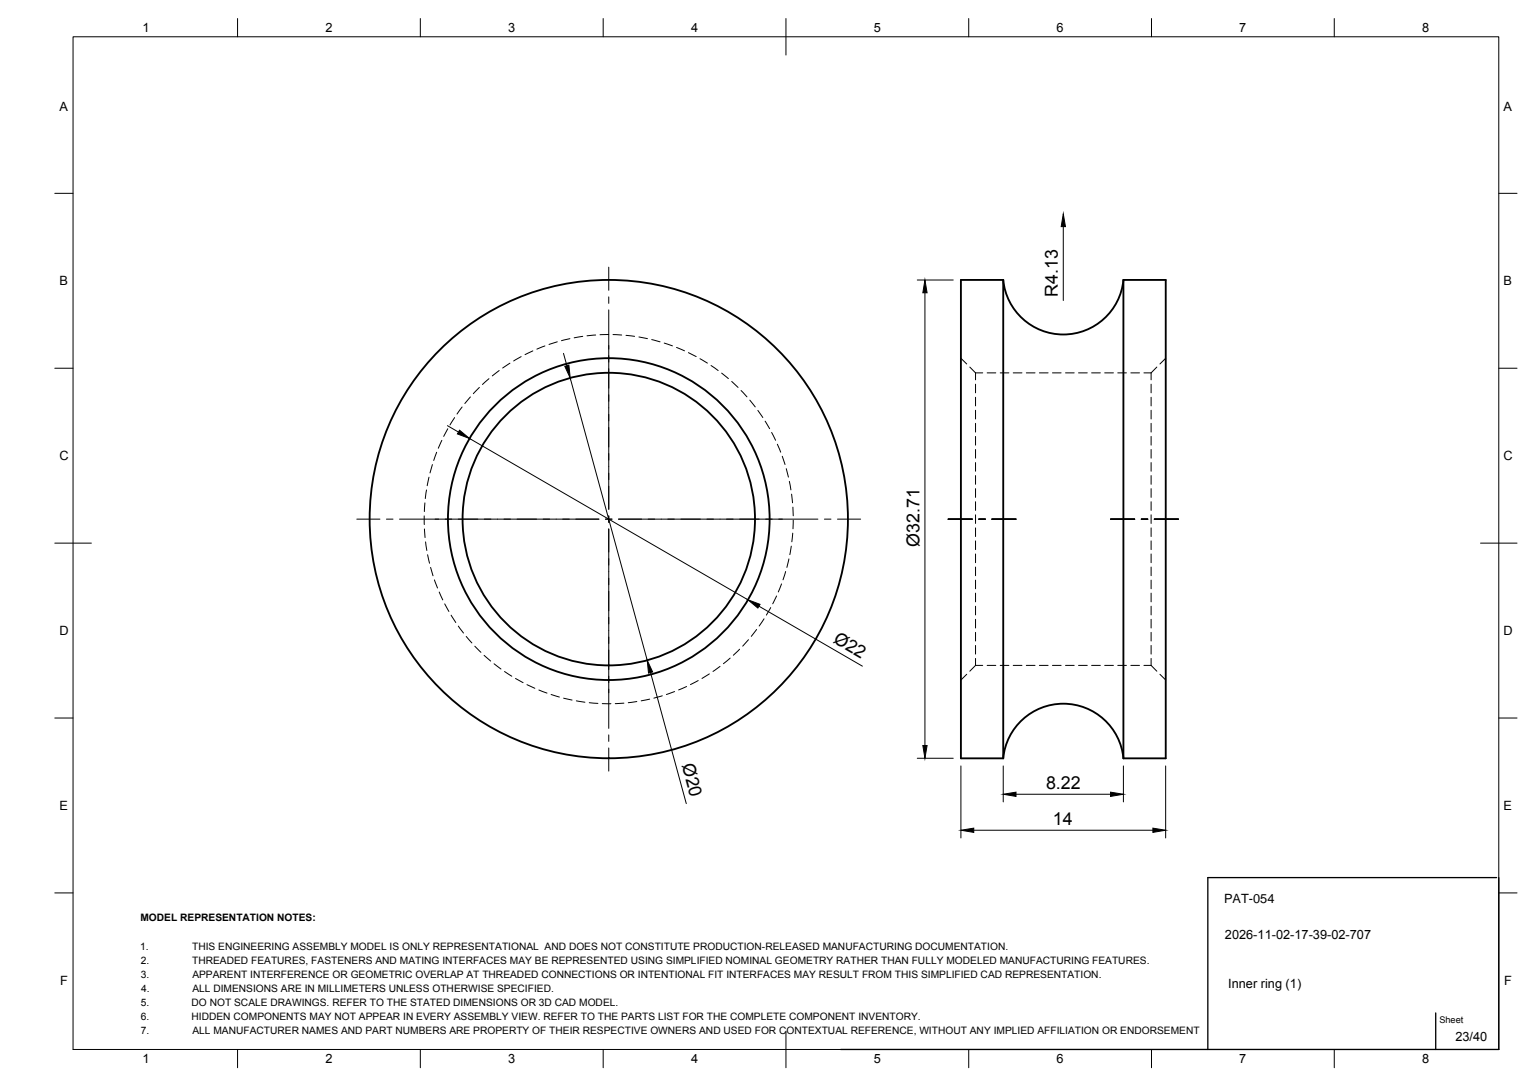
ISO-10303-21;
HEADER;
/* Generated by software containing ST-Developer
 * from STEP Tools, Inc. (www.steptools.com) 
 */

FILE_DESCRIPTION(
/* description */ ('PAT-054'),
/* implementation_level */ '2;1');

FILE_NAME(
/* name */ 'Inner ring (1).step',
/* time_stamp */ '2026-10-29T16:38:13-07:00',
/* author */ (''),
/* organization */ (''),
/* preprocessor_version */ 'ST-DEVELOPER v20.2',
/* originating_system */ 'Autodesk Translation Framework v15.17.0.0',
/* authorisation */ '');

FILE_SCHEMA (('AUTOMOTIVE_DESIGN { 1 0 10303 214 3 1 1 }'));
ENDSEC;

DATA;
#10=MECHANICAL_DESIGN_GEOMETRIC_PRESENTATION_REPRESENTATION('',(#920),#33981);
#781=CONICAL_SURFACE('',#14012,1.05,0.785398163397449);
#782=CONICAL_SURFACE('',#14019,1.05,0.785398163397449);
#809=TOROIDAL_SURFACE('',#14001,1.675,0.412776);
#825=SHAPE_REPRESENTATION_RELATIONSHIP('SRR','None',#34200,#869);
#869=ADVANCED_BREP_SHAPE_REPRESENTATION('',(#979),#33948);
#920=STYLED_ITEM('',(#34517),#979);
#979=MANIFOLD_SOLID_BREP('Body1',#13031);
#1137=FACE_BOUND('',#2629,.T.);
#1138=FACE_BOUND('',#2632,.T.);
#1327=PLANE('',#14014);
#1328=PLANE('',#14017);
#1776=FACE_OUTER_BOUND('',#2624,.T.);
#1777=FACE_OUTER_BOUND('',#2625,.T.);
#1778=FACE_OUTER_BOUND('',#2626,.T.);
#1779=FACE_OUTER_BOUND('',#2627,.T.);
#1780=FACE_OUTER_BOUND('',#2628,.T.);
#1781=FACE_OUTER_BOUND('',#2630,.T.);
#1782=FACE_OUTER_BOUND('',#2631,.T.);
#1783=FACE_OUTER_BOUND('',#2633,.T.);
#2624=EDGE_LOOP('',(#9425,#9426,#9427,#9428,#9429,#9430));
#2625=EDGE_LOOP('',(#9431,#9432,#9433,#9434,#9435));
#2626=EDGE_LOOP('',(#9436,#9437,#9438,#9439));
#2627=EDGE_LOOP('',(#9440,#9441,#9442,#9443));
#2628=EDGE_LOOP('',(#9444));
#2629=EDGE_LOOP('',(#9445));
#2630=EDGE_LOOP('',(#9446,#9447,#9448,#9449,#9450));
#2631=EDGE_LOOP('',(#9451));
#2632=EDGE_LOOP('',(#9452));
#2633=EDGE_LOOP('',(#9453,#9454,#9455,#9456));
#3474=LINE('',#19805,#4408);
#3475=LINE('',#19811,#4409);
#3476=LINE('',#19815,#4410);
#3477=LINE('',#19821,#4411);
#3478=LINE('',#19826,#4412);
#4408=VECTOR('',#16025,1.63531);
#4409=VECTOR('',#16032,1.);
#4410=VECTOR('',#16037,1.05);
#4411=VECTOR('',#16046,1.63531);
#4412=VECTOR('',#16053,1.05);
#5322=CIRCLE('',#14002,1.63531);
#5323=CIRCLE('',#14003,1.63531);
#5324=CIRCLE('',#14004,0.412776);
#5325=CIRCLE('',#14005,1.63531);
#5326=CIRCLE('',#14006,1.63531);
#5327=CIRCLE('',#14008,1.63531);
#5328=CIRCLE('',#14010,1.);
#5329=CIRCLE('',#14011,1.);
#5330=CIRCLE('',#14013,1.1);
#5331=CIRCLE('',#14016,1.63531);
#5332=CIRCLE('',#14018,1.1);
#5890=VERTEX_POINT('',#19794);
#5891=VERTEX_POINT('',#19795);
#5892=VERTEX_POINT('',#19798);
#5893=VERTEX_POINT('',#19800);
#5894=VERTEX_POINT('',#19804);
#5895=VERTEX_POINT('',#19808);
#5896=VERTEX_POINT('',#19810);
#5897=VERTEX_POINT('',#19814);
#5898=VERTEX_POINT('',#19819);
#5899=VERTEX_POINT('',#19823);
#7212=EDGE_CURVE('',#5890,#5891,#5322,.T.);
#7213=EDGE_CURVE('',#5891,#5890,#5323,.T.);
#7214=EDGE_CURVE('',#5891,#5892,#5324,.T.);
#7215=EDGE_CURVE('',#5893,#5892,#5325,.T.);
#7216=EDGE_CURVE('',#5892,#5893,#5326,.T.);
#7217=EDGE_CURVE('',#5893,#5894,#3474,.T.);
#7218=EDGE_CURVE('',#5894,#5894,#5327,.T.);
#7219=EDGE_CURVE('',#5895,#5895,#5328,.T.);
#7220=EDGE_CURVE('',#5895,#5896,#3475,.T.);
#7221=EDGE_CURVE('',#5896,#5896,#5329,.T.);
#7222=EDGE_CURVE('',#5896,#5897,#3476,.T.);
#7223=EDGE_CURVE('',#5897,#5897,#5330,.T.);
#7224=EDGE_CURVE('',#5898,#5898,#5331,.T.);
#7225=EDGE_CURVE('',#5898,#5890,#3477,.T.);
#7226=EDGE_CURVE('',#5899,#5899,#5332,.T.);
#7227=EDGE_CURVE('',#5899,#5895,#3478,.T.);
#9425=ORIENTED_EDGE('',*,*,#7212,.F.);
#9426=ORIENTED_EDGE('',*,*,#7213,.F.);
#9427=ORIENTED_EDGE('',*,*,#7214,.T.);
#9428=ORIENTED_EDGE('',*,*,#7215,.F.);
#9429=ORIENTED_EDGE('',*,*,#7216,.F.);
#9430=ORIENTED_EDGE('',*,*,#7214,.F.);
#9431=ORIENTED_EDGE('',*,*,#7215,.T.);
#9432=ORIENTED_EDGE('',*,*,#7216,.T.);
#9433=ORIENTED_EDGE('',*,*,#7217,.T.);
#9434=ORIENTED_EDGE('',*,*,#7218,.T.);
#9435=ORIENTED_EDGE('',*,*,#7217,.F.);
#9436=ORIENTED_EDGE('',*,*,#7219,.T.);
#9437=ORIENTED_EDGE('',*,*,#7220,.T.);
#9438=ORIENTED_EDGE('',*,*,#7221,.F.);
#9439=ORIENTED_EDGE('',*,*,#7220,.F.);
#9440=ORIENTED_EDGE('',*,*,#7221,.T.);
#9441=ORIENTED_EDGE('',*,*,#7222,.T.);
#9442=ORIENTED_EDGE('',*,*,#7223,.F.);
#9443=ORIENTED_EDGE('',*,*,#7222,.F.);
#9444=ORIENTED_EDGE('',*,*,#7218,.F.);
#9445=ORIENTED_EDGE('',*,*,#7223,.T.);
#9446=ORIENTED_EDGE('',*,*,#7224,.F.);
#9447=ORIENTED_EDGE('',*,*,#7225,.T.);
#9448=ORIENTED_EDGE('',*,*,#7212,.T.);
#9449=ORIENTED_EDGE('',*,*,#7213,.T.);
#9450=ORIENTED_EDGE('',*,*,#7225,.F.);
#9451=ORIENTED_EDGE('',*,*,#7224,.T.);
#9452=ORIENTED_EDGE('',*,*,#7226,.F.);
#9453=ORIENTED_EDGE('',*,*,#7226,.T.);
#9454=ORIENTED_EDGE('',*,*,#7227,.T.);
#9455=ORIENTED_EDGE('',*,*,#7219,.F.);
#9456=ORIENTED_EDGE('',*,*,#7227,.F.);
#12061=CYLINDRICAL_SURFACE('',#14007,1.63531);
#12062=CYLINDRICAL_SURFACE('',#14009,1.);
#12063=CYLINDRICAL_SURFACE('',#14015,1.63531);
#12488=ADVANCED_FACE('',(#1776),#809,.F.);
#12489=ADVANCED_FACE('',(#1777),#12061,.T.);
#12490=ADVANCED_FACE('',(#1778),#12062,.F.);
#12491=ADVANCED_FACE('',(#1779),#781,.F.);
#12492=ADVANCED_FACE('',(#1780,#1137),#1327,.T.);
#12493=ADVANCED_FACE('',(#1781),#12063,.T.);
#12494=ADVANCED_FACE('',(#1782,#1138),#1328,.T.);
#12495=ADVANCED_FACE('',(#1783),#782,.F.);
#13031=CLOSED_SHELL('',(#12488,#12489,#12490,#12491,#12492,#12493,#12494,
#12495));
#14000=AXIS2_PLACEMENT_3D('',#19792,#16009,#16010);
#14001=AXIS2_PLACEMENT_3D('',#19793,#16011,#16012);
#14002=AXIS2_PLACEMENT_3D('',#19796,#16013,#16014);
#14003=AXIS2_PLACEMENT_3D('',#19797,#16015,#16016);
#14004=AXIS2_PLACEMENT_3D('',#19799,#16017,#16018);
#14005=AXIS2_PLACEMENT_3D('',#19801,#16019,#16020);
#14006=AXIS2_PLACEMENT_3D('',#19802,#16021,#16022);
#14007=AXIS2_PLACEMENT_3D('',#19803,#16023,#16024);
#14008=AXIS2_PLACEMENT_3D('',#19806,#16026,#16027);
#14009=AXIS2_PLACEMENT_3D('',#19807,#16028,#16029);
#14010=AXIS2_PLACEMENT_3D('',#19809,#16030,#16031);
#14011=AXIS2_PLACEMENT_3D('',#19812,#16033,#16034);
#14012=AXIS2_PLACEMENT_3D('',#19813,#16035,#16036);
#14013=AXIS2_PLACEMENT_3D('',#19816,#16038,#16039);
#14014=AXIS2_PLACEMENT_3D('',#19817,#16040,#16041);
#14015=AXIS2_PLACEMENT_3D('',#19818,#16042,#16043);
#14016=AXIS2_PLACEMENT_3D('',#19820,#16044,#16045);
#14017=AXIS2_PLACEMENT_3D('',#19822,#16047,#16048);
#14018=AXIS2_PLACEMENT_3D('',#19824,#16049,#16050);
#14019=AXIS2_PLACEMENT_3D('',#19825,#16051,#16052);
#16009=DIRECTION('axis',(0.,0.,1.));
#16010=DIRECTION('refdir',(1.,0.,0.));
#16011=DIRECTION('center_axis',(0.,-1.,0.));
#16012=DIRECTION('ref_axis',(0.,0.,-1.));
#16013=DIRECTION('center_axis',(0.,-1.,0.));
#16014=DIRECTION('ref_axis',(1.,0.,0.));
#16015=DIRECTION('center_axis',(0.,-1.,0.));
#16016=DIRECTION('ref_axis',(1.,0.,0.));
#16017=DIRECTION('center_axis',(1.,0.,1.22464679914735E-16));
#16018=DIRECTION('ref_axis',(-1.22464679914735E-16,0.,1.));
#16019=DIRECTION('center_axis',(0.,1.,0.));
#16020=DIRECTION('ref_axis',(1.,0.,0.));
#16021=DIRECTION('center_axis',(0.,1.,0.));
#16022=DIRECTION('ref_axis',(1.,0.,0.));
#16023=DIRECTION('center_axis',(0.,-1.,0.));
#16024=DIRECTION('ref_axis',(1.,0.,0.));
#16025=DIRECTION('',(0.,1.,0.));
#16026=DIRECTION('center_axis',(0.,-1.,0.));
#16027=DIRECTION('ref_axis',(1.,0.,0.));
#16028=DIRECTION('center_axis',(0.,-1.,0.));
#16029=DIRECTION('ref_axis',(1.,0.,0.));
#16030=DIRECTION('center_axis',(0.,-1.,0.));
#16031=DIRECTION('ref_axis',(1.,0.,0.));
#16032=DIRECTION('',(0.,1.,0.));
#16033=DIRECTION('center_axis',(0.,-1.,0.));
#16034=DIRECTION('ref_axis',(1.,0.,0.));
#16035=DIRECTION('center_axis',(0.,1.,0.));
#16036=DIRECTION('ref_axis',(1.,0.,0.));
#16037=DIRECTION('',(-0.707106781186548,0.707106781186547,-8.65956056235494E-17));
#16038=DIRECTION('center_axis',(0.,-1.,0.));
#16039=DIRECTION('ref_axis',(1.,0.,0.));
#16040=DIRECTION('center_axis',(0.,1.,0.));
#16041=DIRECTION('ref_axis',(0.,0.,1.));
#16042=DIRECTION('center_axis',(0.,-1.,0.));
#16043=DIRECTION('ref_axis',(1.,0.,0.));
#16044=DIRECTION('center_axis',(0.,-1.,0.));
#16045=DIRECTION('ref_axis',(1.,0.,0.));
#16046=DIRECTION('',(0.,1.,0.));
#16047=DIRECTION('center_axis',(0.,-1.,0.));
#16048=DIRECTION('ref_axis',(0.,0.,-1.));
#16049=DIRECTION('center_axis',(0.,-1.,0.));
#16050=DIRECTION('ref_axis',(1.,0.,0.));
#16051=DIRECTION('center_axis',(0.,-1.,0.));
#16052=DIRECTION('ref_axis',(1.,0.,0.));
#16053=DIRECTION('',(0.707106781186548,0.707106781186547,8.65956056235494E-17));
#19792=CARTESIAN_POINT('',(0.,0.,0.));
#19793=CARTESIAN_POINT('Origin',(0.,0.,0.));
#19794=CARTESIAN_POINT('',(-1.63531,-0.410863395882378,-2.00267715711366E-16));
#19795=CARTESIAN_POINT('',(-2.00267715711366E-16,-0.410863395882378,1.63531));
#19796=CARTESIAN_POINT('Origin',(0.,-0.410863395882378,0.));
#19797=CARTESIAN_POINT('Origin',(0.,-0.410863395882378,0.));
#19798=CARTESIAN_POINT('',(-2.00267715711366E-16,0.410863395882378,1.63531));
#19799=CARTESIAN_POINT('Origin',(-2.05128338857182E-16,0.,1.675));
#19800=CARTESIAN_POINT('',(-1.63531,0.410863395882378,2.00267715711366E-16));
#19801=CARTESIAN_POINT('Origin',(0.,0.410863395882378,0.));
#19802=CARTESIAN_POINT('Origin',(0.,0.410863395882378,0.));
#19803=CARTESIAN_POINT('Origin',(0.,0.,0.));
#19804=CARTESIAN_POINT('',(-1.63531,0.7,-2.00267715711366E-16));
#19805=CARTESIAN_POINT('',(-1.63531,0.,-2.00267715711366E-16));
#19806=CARTESIAN_POINT('Origin',(0.,0.7,0.));
#19807=CARTESIAN_POINT('Origin',(0.,0.,0.));
#19808=CARTESIAN_POINT('',(-1.,-0.6,-1.22464679914735E-16));
#19809=CARTESIAN_POINT('Origin',(0.,-0.6,0.));
#19810=CARTESIAN_POINT('',(-1.,0.6,-1.22464679914735E-16));
#19811=CARTESIAN_POINT('',(-1.,0.,-1.22464679914735E-16));
#19812=CARTESIAN_POINT('Origin',(0.,0.6,0.));
#19813=CARTESIAN_POINT('Origin',(0.,0.65,0.));
#19814=CARTESIAN_POINT('',(-1.1,0.7,-1.34711147906209E-16));
#19815=CARTESIAN_POINT('',(-1.05,0.65,-1.28587913910472E-16));
#19816=CARTESIAN_POINT('Origin',(0.,0.7,0.));
#19817=CARTESIAN_POINT('Origin',(1.63531,0.7,0.));
#19818=CARTESIAN_POINT('Origin',(0.,0.,0.));
#19819=CARTESIAN_POINT('',(-1.63531,-0.7,-2.00267715711366E-16));
#19820=CARTESIAN_POINT('Origin',(0.,-0.7,0.));
#19821=CARTESIAN_POINT('',(-1.63531,0.,-2.00267715711366E-16));
#19822=CARTESIAN_POINT('Origin',(1.1,-0.7,0.));
#19823=CARTESIAN_POINT('',(-1.1,-0.7,-1.34711147906209E-16));
#19824=CARTESIAN_POINT('Origin',(0.,-0.7,0.));
#19825=CARTESIAN_POINT('Origin',(0.,-0.65,0.));
#19826=CARTESIAN_POINT('',(-1.05,-0.65,-1.28587913910472E-16));
#33896=UNCERTAINTY_MEASURE_WITH_UNIT(LENGTH_MEASURE(0.001),#33982,
'DISTANCE_ACCURACY_VALUE',
'Maximum model space distance between geometric entities at asserted c
onnectivities');
#33929=UNCERTAINTY_MEASURE_WITH_UNIT(LENGTH_MEASURE(0.001),#33982,
'DISTANCE_ACCURACY_VALUE',
'Maximum model space distance between geometric entities at asserted c
onnectivities');
#33948=(
GEOMETRIC_REPRESENTATION_CONTEXT(3)
GLOBAL_UNCERTAINTY_ASSIGNED_CONTEXT((#33896))
GLOBAL_UNIT_ASSIGNED_CONTEXT((#33982,#33984,#33985))
REPRESENTATION_CONTEXT('','3D')
);
#33981=(
GEOMETRIC_REPRESENTATION_CONTEXT(3)
GLOBAL_UNCERTAINTY_ASSIGNED_CONTEXT((#33929))
GLOBAL_UNIT_ASSIGNED_CONTEXT((#33982,#33984,#33985))
REPRESENTATION_CONTEXT('','3D')
);
#33982=(
LENGTH_UNIT()
NAMED_UNIT(*)
SI_UNIT(.CENTI.,.METRE.)
);
#33984=(
NAMED_UNIT(*)
PLANE_ANGLE_UNIT()
SI_UNIT($,.RADIAN.)
);
#33985=(
NAMED_UNIT(*)
SI_UNIT($,.STERADIAN.)
SOLID_ANGLE_UNIT()
);
#34004=SHAPE_DEFINITION_REPRESENTATION(#34060,#34200);
#34060=PRODUCT_DEFINITION_SHAPE('',$,#34252);
#34200=SHAPE_REPRESENTATION('',(#14000),#33948);
#34233=PRODUCT_DEFINITION_CONTEXT('part definition',#34388,'design');
#34252=PRODUCT_DEFINITION('Inner ring (1)','Inner ring (1)',#34303,#34233);
#34303=PRODUCT_DEFINITION_FORMATION('',$,#34408);
#34388=APPLICATION_CONTEXT(
'Core Data for Automotive Mechanical Design Process');
#34389=PRODUCT_CONTEXT('part definition',#34388,'mechanical');
#34408=PRODUCT('Inner ring (1)','Inner ring (1)','Inner ring (1)',(#34389));
#34511=COLOUR_RGB('Grey',0.48,0.52,0.57);
#34512=FILL_AREA_STYLE_COLOUR('',#34511);
#34513=FILL_AREA_STYLE('',(#34512));
#34514=SURFACE_STYLE_FILL_AREA(#34513);
#34515=SURFACE_SIDE_STYLE('',(#34514));
#34516=SURFACE_STYLE_USAGE(.BOTH.,#34515);
#34517=PRESENTATION_STYLE_ASSIGNMENT((#34516));
ENDSEC;
END-ISO-10303-21;
